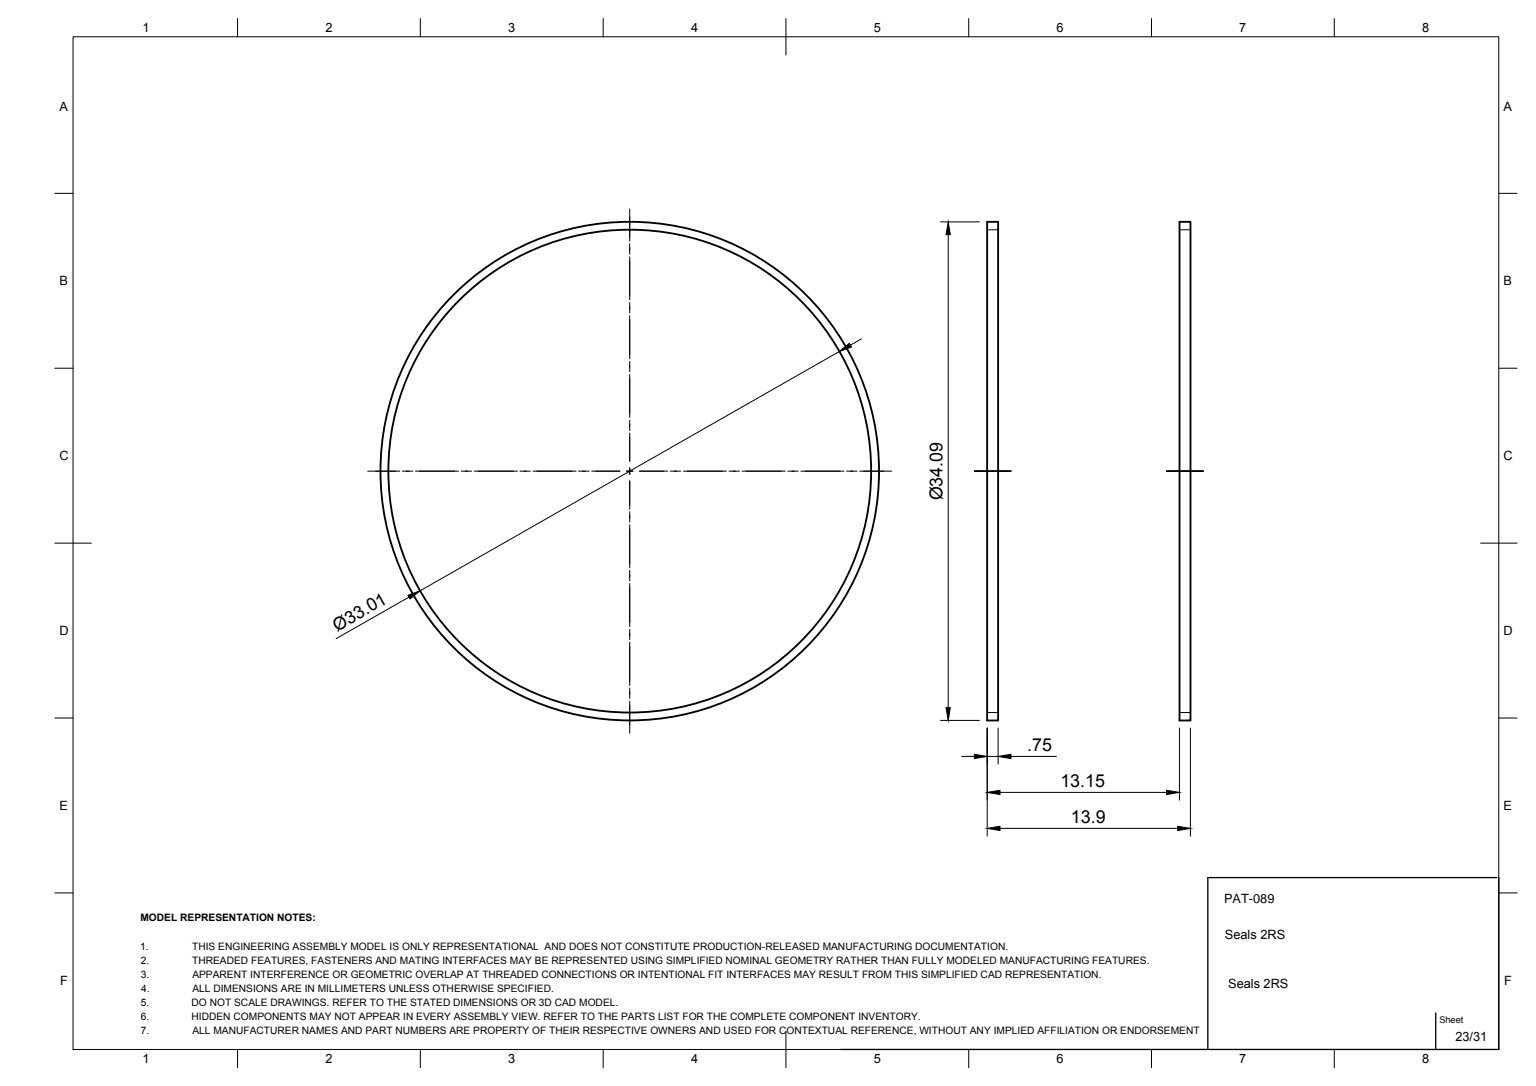
ISO-10303-21;
HEADER;
/* Generated by software containing ST-Developer
 * from STEP Tools, Inc. (www.steptools.com) 
 */

FILE_DESCRIPTION(
/* description */ ('Rotary union on bearing shaft'),
/* implementation_level */ '2;1');

FILE_NAME(
/* name */ 'Seals 2RS.step',
/* time_stamp */ '2026-10-28T03:24:01-07:00',
/* author */ (''),
/* organization */ (''),
/* preprocessor_version */ 'ST-DEVELOPER v20.2',
/* originating_system */ 'Autodesk Translation Framework v15.17.0.0',
/* authorisation */ '');

FILE_SCHEMA (('AUTOMOTIVE_DESIGN { 1 0 10303 214 3 1 1 }'));
ENDSEC;

DATA;
#10=MECHANICAL_DESIGN_GEOMETRIC_PRESENTATION_REPRESENTATION('',(#335,#336),#9448);
#274=SHAPE_REPRESENTATION_RELATIONSHIP('SRR','None',#9575,#301);
#301=ADVANCED_BREP_SHAPE_REPRESENTATION('',(#370,#371),#9435);
#335=STYLED_ITEM('',(#9778),#370);
#336=STYLED_ITEM('',(#9778),#371);
#370=MANIFOLD_SOLID_BREP('Body1',#4890);
#371=MANIFOLD_SOLID_BREP('Body2',#4891);
#449=FACE_BOUND('',#1179,.T.);
#450=FACE_BOUND('',#1182,.T.);
#451=FACE_BOUND('',#1185,.T.);
#452=FACE_BOUND('',#1188,.T.);
#563=PLANE('',#5540);
#564=PLANE('',#5545);
#565=PLANE('',#5548);
#566=PLANE('',#5553);
#810=FACE_OUTER_BOUND('',#1178,.T.);
#811=FACE_OUTER_BOUND('',#1180,.T.);
#812=FACE_OUTER_BOUND('',#1181,.T.);
#813=FACE_OUTER_BOUND('',#1183,.T.);
#814=FACE_OUTER_BOUND('',#1184,.T.);
#815=FACE_OUTER_BOUND('',#1186,.T.);
#816=FACE_OUTER_BOUND('',#1187,.T.);
#817=FACE_OUTER_BOUND('',#1189,.T.);
#1178=EDGE_LOOP('',(#3911));
#1179=EDGE_LOOP('',(#3912));
#1180=EDGE_LOOP('',(#3913,#3914,#3915,#3916));
#1181=EDGE_LOOP('',(#3917));
#1182=EDGE_LOOP('',(#3918));
#1183=EDGE_LOOP('',(#3919,#3920,#3921,#3922));
#1184=EDGE_LOOP('',(#3923));
#1185=EDGE_LOOP('',(#3924));
#1186=EDGE_LOOP('',(#3925,#3926,#3927,#3928));
#1187=EDGE_LOOP('',(#3929));
#1188=EDGE_LOOP('',(#3930));
#1189=EDGE_LOOP('',(#3931,#3932,#3933,#3934));
#1494=LINE('',#8589,#1814);
#1495=LINE('',#8594,#1815);
#1496=LINE('',#8603,#1816);
#1497=LINE('',#8608,#1817);
#1814=VECTOR('',#6643,1.70469);
#1815=VECTOR('',#6650,1.65031);
#1816=VECTOR('',#6661,1.70469);
#1817=VECTOR('',#6668,1.65031);
#2164=CIRCLE('',#5541,1.70469);
#2165=CIRCLE('',#5542,1.65031);
#2166=CIRCLE('',#5544,1.70469);
#2167=CIRCLE('',#5546,1.65031);
#2168=CIRCLE('',#5549,1.70469);
#2169=CIRCLE('',#5550,1.65031);
#2170=CIRCLE('',#5552,1.70469);
#2171=CIRCLE('',#5554,1.65031);
#2476=VERTEX_POINT('',#8582);
#2477=VERTEX_POINT('',#8584);
#2478=VERTEX_POINT('',#8587);
#2479=VERTEX_POINT('',#8591);
#2480=VERTEX_POINT('',#8596);
#2481=VERTEX_POINT('',#8598);
#2482=VERTEX_POINT('',#8601);
#2483=VERTEX_POINT('',#8605);
#2983=EDGE_CURVE('',#2476,#2476,#2164,.T.);
#2984=EDGE_CURVE('',#2477,#2477,#2165,.T.);
#2985=EDGE_CURVE('',#2478,#2478,#2166,.T.);
#2986=EDGE_CURVE('',#2478,#2476,#1494,.T.);
#2987=EDGE_CURVE('',#2479,#2479,#2167,.T.);
#2988=EDGE_CURVE('',#2479,#2477,#1495,.T.);
#2989=EDGE_CURVE('',#2480,#2480,#2168,.T.);
#2990=EDGE_CURVE('',#2481,#2481,#2169,.T.);
#2991=EDGE_CURVE('',#2482,#2482,#2170,.T.);
#2992=EDGE_CURVE('',#2482,#2480,#1496,.T.);
#2993=EDGE_CURVE('',#2483,#2483,#2171,.T.);
#2994=EDGE_CURVE('',#2483,#2481,#1497,.T.);
#3911=ORIENTED_EDGE('',*,*,#2983,.F.);
#3912=ORIENTED_EDGE('',*,*,#2984,.T.);
#3913=ORIENTED_EDGE('',*,*,#2985,.F.);
#3914=ORIENTED_EDGE('',*,*,#2986,.T.);
#3915=ORIENTED_EDGE('',*,*,#2983,.T.);
#3916=ORIENTED_EDGE('',*,*,#2986,.F.);
#3917=ORIENTED_EDGE('',*,*,#2985,.T.);
#3918=ORIENTED_EDGE('',*,*,#2987,.F.);
#3919=ORIENTED_EDGE('',*,*,#2987,.T.);
#3920=ORIENTED_EDGE('',*,*,#2988,.T.);
#3921=ORIENTED_EDGE('',*,*,#2984,.F.);
#3922=ORIENTED_EDGE('',*,*,#2988,.F.);
#3923=ORIENTED_EDGE('',*,*,#2989,.F.);
#3924=ORIENTED_EDGE('',*,*,#2990,.T.);
#3925=ORIENTED_EDGE('',*,*,#2991,.F.);
#3926=ORIENTED_EDGE('',*,*,#2992,.T.);
#3927=ORIENTED_EDGE('',*,*,#2989,.T.);
#3928=ORIENTED_EDGE('',*,*,#2992,.F.);
#3929=ORIENTED_EDGE('',*,*,#2991,.T.);
#3930=ORIENTED_EDGE('',*,*,#2993,.F.);
#3931=ORIENTED_EDGE('',*,*,#2993,.T.);
#3932=ORIENTED_EDGE('',*,*,#2994,.T.);
#3933=ORIENTED_EDGE('',*,*,#2990,.F.);
#3934=ORIENTED_EDGE('',*,*,#2994,.F.);
#4533=CYLINDRICAL_SURFACE('',#5543,1.70469);
#4534=CYLINDRICAL_SURFACE('',#5547,1.65031);
#4535=CYLINDRICAL_SURFACE('',#5551,1.70469);
#4536=CYLINDRICAL_SURFACE('',#5555,1.65031);
#4723=ADVANCED_FACE('',(#810,#449),#563,.T.);
#4724=ADVANCED_FACE('',(#811),#4533,.T.);
#4725=ADVANCED_FACE('',(#812,#450),#564,.T.);
#4726=ADVANCED_FACE('',(#813),#4534,.F.);
#4727=ADVANCED_FACE('',(#814,#451),#565,.T.);
#4728=ADVANCED_FACE('',(#815),#4535,.T.);
#4729=ADVANCED_FACE('',(#816,#452),#566,.T.);
#4730=ADVANCED_FACE('',(#817),#4536,.F.);
#4890=CLOSED_SHELL('',(#4723,#4724,#4725,#4726));
#4891=CLOSED_SHELL('',(#4727,#4728,#4729,#4730));
#5539=AXIS2_PLACEMENT_3D('',#8580,#6631,#6632);
#5540=AXIS2_PLACEMENT_3D('',#8581,#6633,#6634);
#5541=AXIS2_PLACEMENT_3D('',#8583,#6635,#6636);
#5542=AXIS2_PLACEMENT_3D('',#8585,#6637,#6638);
#5543=AXIS2_PLACEMENT_3D('',#8586,#6639,#6640);
#5544=AXIS2_PLACEMENT_3D('',#8588,#6641,#6642);
#5545=AXIS2_PLACEMENT_3D('',#8590,#6644,#6645);
#5546=AXIS2_PLACEMENT_3D('',#8592,#6646,#6647);
#5547=AXIS2_PLACEMENT_3D('',#8593,#6648,#6649);
#5548=AXIS2_PLACEMENT_3D('',#8595,#6651,#6652);
#5549=AXIS2_PLACEMENT_3D('',#8597,#6653,#6654);
#5550=AXIS2_PLACEMENT_3D('',#8599,#6655,#6656);
#5551=AXIS2_PLACEMENT_3D('',#8600,#6657,#6658);
#5552=AXIS2_PLACEMENT_3D('',#8602,#6659,#6660);
#5553=AXIS2_PLACEMENT_3D('',#8604,#6662,#6663);
#5554=AXIS2_PLACEMENT_3D('',#8606,#6664,#6665);
#5555=AXIS2_PLACEMENT_3D('',#8607,#6666,#6667);
#6631=DIRECTION('axis',(0.,0.,1.));
#6632=DIRECTION('refdir',(1.,0.,0.));
#6633=DIRECTION('center_axis',(0.,1.,0.));
#6634=DIRECTION('ref_axis',(0.,0.,1.));
#6635=DIRECTION('center_axis',(0.,-1.,0.));
#6636=DIRECTION('ref_axis',(1.,0.,0.));
#6637=DIRECTION('center_axis',(0.,-1.,0.));
#6638=DIRECTION('ref_axis',(1.,0.,0.));
#6639=DIRECTION('center_axis',(0.,-1.,0.));
#6640=DIRECTION('ref_axis',(1.,0.,0.));
#6641=DIRECTION('center_axis',(0.,-1.,0.));
#6642=DIRECTION('ref_axis',(1.,0.,0.));
#6643=DIRECTION('',(0.,1.,0.));
#6644=DIRECTION('center_axis',(0.,-1.,0.));
#6645=DIRECTION('ref_axis',(0.,0.,-1.));
#6646=DIRECTION('center_axis',(0.,-1.,0.));
#6647=DIRECTION('ref_axis',(1.,0.,0.));
#6648=DIRECTION('center_axis',(0.,-1.,0.));
#6649=DIRECTION('ref_axis',(1.,0.,0.));
#6650=DIRECTION('',(0.,1.,0.));
#6651=DIRECTION('center_axis',(0.,1.,0.));
#6652=DIRECTION('ref_axis',(0.,0.,1.));
#6653=DIRECTION('center_axis',(0.,-1.,0.));
#6654=DIRECTION('ref_axis',(1.,0.,0.));
#6655=DIRECTION('center_axis',(0.,-1.,0.));
#6656=DIRECTION('ref_axis',(1.,0.,0.));
#6657=DIRECTION('center_axis',(0.,-1.,0.));
#6658=DIRECTION('ref_axis',(1.,0.,0.));
#6659=DIRECTION('center_axis',(0.,-1.,0.));
#6660=DIRECTION('ref_axis',(1.,0.,0.));
#6661=DIRECTION('',(0.,1.,0.));
#6662=DIRECTION('center_axis',(0.,-1.,0.));
#6663=DIRECTION('ref_axis',(0.,0.,-1.));
#6664=DIRECTION('center_axis',(0.,-1.,0.));
#6665=DIRECTION('ref_axis',(1.,0.,0.));
#6666=DIRECTION('center_axis',(0.,-1.,0.));
#6667=DIRECTION('ref_axis',(1.,0.,0.));
#6668=DIRECTION('',(0.,1.,0.));
#8580=CARTESIAN_POINT('',(0.,0.,0.));
#8581=CARTESIAN_POINT('Origin',(1.70469,0.695,0.));
#8582=CARTESIAN_POINT('',(-1.70469,0.695,-2.0876431520385E-16));
#8583=CARTESIAN_POINT('Origin',(0.,0.695,0.));
#8584=CARTESIAN_POINT('',(-1.65031,0.695,-2.02104685910087E-16));
#8585=CARTESIAN_POINT('Origin',(0.,0.695,0.));
#8586=CARTESIAN_POINT('Origin',(0.,0.6575,0.));
#8587=CARTESIAN_POINT('',(-1.70469,0.62,-2.0876431520385E-16));
#8588=CARTESIAN_POINT('Origin',(0.,0.62,0.));
#8589=CARTESIAN_POINT('',(-1.70469,0.6575,-2.0876431520385E-16));
#8590=CARTESIAN_POINT('Origin',(1.65031,0.62,0.));
#8591=CARTESIAN_POINT('',(-1.65031,0.62,-2.02104685910087E-16));
#8592=CARTESIAN_POINT('Origin',(0.,0.62,0.));
#8593=CARTESIAN_POINT('Origin',(0.,0.6575,0.));
#8594=CARTESIAN_POINT('',(-1.65031,0.6575,-2.02104685910087E-16));
#8595=CARTESIAN_POINT('Origin',(1.70469,-0.62,0.));
#8596=CARTESIAN_POINT('',(-1.70469,-0.62,-2.0876431520385E-16));
#8597=CARTESIAN_POINT('Origin',(0.,-0.62,0.));
#8598=CARTESIAN_POINT('',(-1.65031,-0.62,-2.02104685910087E-16));
#8599=CARTESIAN_POINT('Origin',(0.,-0.62,0.));
#8600=CARTESIAN_POINT('Origin',(0.,-0.6575,0.));
#8601=CARTESIAN_POINT('',(-1.70469,-0.695,-2.0876431520385E-16));
#8602=CARTESIAN_POINT('Origin',(0.,-0.695,0.));
#8603=CARTESIAN_POINT('',(-1.70469,-0.6575,-2.0876431520385E-16));
#8604=CARTESIAN_POINT('Origin',(1.65031,-0.695,0.));
#8605=CARTESIAN_POINT('',(-1.65031,-0.695,-2.02104685910087E-16));
#8606=CARTESIAN_POINT('Origin',(0.,-0.695,0.));
#8607=CARTESIAN_POINT('Origin',(0.,-0.6575,0.));
#8608=CARTESIAN_POINT('',(-1.65031,-0.6575,-2.02104685910087E-16));
#9403=UNCERTAINTY_MEASURE_WITH_UNIT(LENGTH_MEASURE(0.001),#9449,
'DISTANCE_ACCURACY_VALUE',
'Maximum model space distance between geometric entities at asserted c
onnectivities');
#9416=UNCERTAINTY_MEASURE_WITH_UNIT(LENGTH_MEASURE(0.001),#9449,
'DISTANCE_ACCURACY_VALUE',
'Maximum model space distance between geometric entities at asserted c
onnectivities');
#9435=(
GEOMETRIC_REPRESENTATION_CONTEXT(3)
GLOBAL_UNCERTAINTY_ASSIGNED_CONTEXT((#9403))
GLOBAL_UNIT_ASSIGNED_CONTEXT((#9449,#9451,#9452))
REPRESENTATION_CONTEXT('','3D')
);
#9448=(
GEOMETRIC_REPRESENTATION_CONTEXT(3)
GLOBAL_UNCERTAINTY_ASSIGNED_CONTEXT((#9416))
GLOBAL_UNIT_ASSIGNED_CONTEXT((#9449,#9451,#9452))
REPRESENTATION_CONTEXT('','3D')
);
#9449=(
LENGTH_UNIT()
NAMED_UNIT(*)
SI_UNIT(.CENTI.,.METRE.)
);
#9451=(
NAMED_UNIT(*)
PLANE_ANGLE_UNIT()
SI_UNIT($,.RADIAN.)
);
#9452=(
NAMED_UNIT(*)
SI_UNIT($,.STERADIAN.)
SOLID_ANGLE_UNIT()
);
#9471=SHAPE_DEFINITION_REPRESENTATION(#9502,#9575);
#9502=PRODUCT_DEFINITION_SHAPE('',$,#9607);
#9575=SHAPE_REPRESENTATION('',(#5539),#9435);
#9588=PRODUCT_DEFINITION_CONTEXT('part definition',#9683,'design');
#9607=PRODUCT_DEFINITION('Seals 2RS','Seals 2RS',#9638,#9588);
#9638=PRODUCT_DEFINITION_FORMATION('',$,#9703);
#9683=APPLICATION_CONTEXT(
'Core Data for Automotive Mechanical Design Process');
#9684=PRODUCT_CONTEXT('part definition',#9683,'mechanical');
#9703=PRODUCT('Seals 2RS','Seals 2RS','Seals 2RS',(#9684));
#9772=COLOUR_RGB('Grey',0.48,0.52,0.57);
#9773=FILL_AREA_STYLE_COLOUR('',#9772);
#9774=FILL_AREA_STYLE('',(#9773));
#9775=SURFACE_STYLE_FILL_AREA(#9774);
#9776=SURFACE_SIDE_STYLE('',(#9775));
#9777=SURFACE_STYLE_USAGE(.BOTH.,#9776);
#9778=PRESENTATION_STYLE_ASSIGNMENT((#9777));
ENDSEC;
END-ISO-10303-21;
